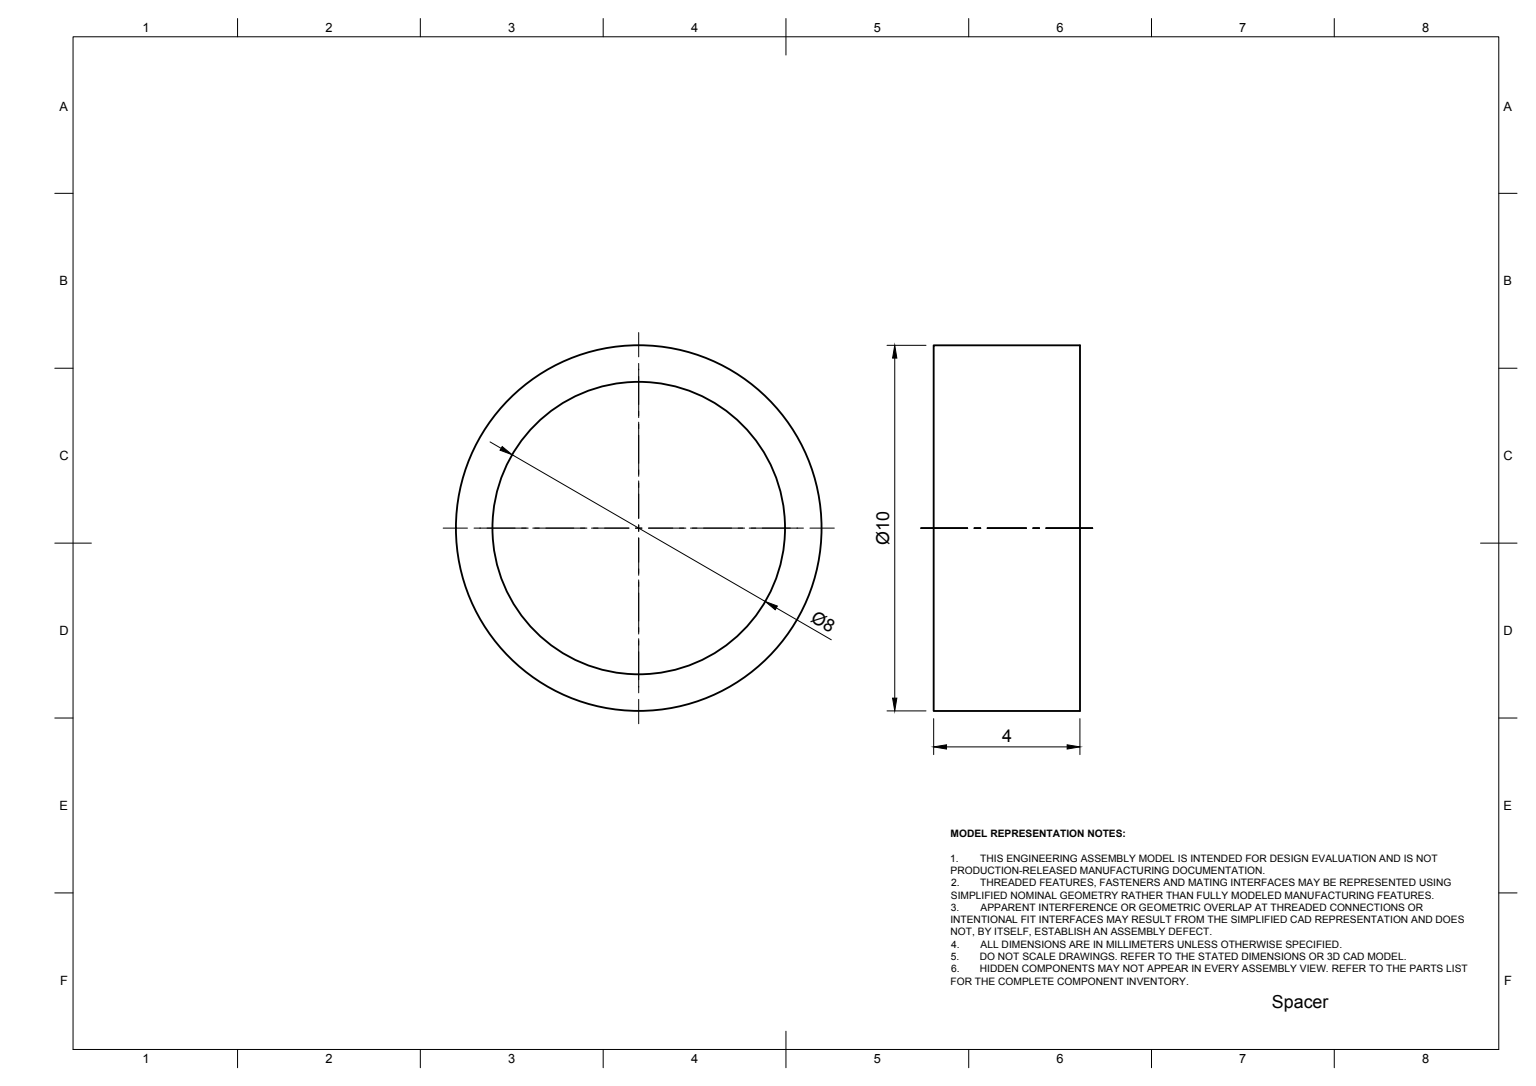
ISO-10303-21;
HEADER;
/* Generated by software containing ST-Developer
 * from STEP Tools, Inc. (www.steptools.com) 
 */

FILE_DESCRIPTION(
/* description */ (''),
/* implementation_level */ '2;1');

FILE_NAME(
/* name */ 'Spacer.step',
/* time_stamp */ '2026-10-04T12:17:52-07:00',
/* author */ (''),
/* organization */ (''),
/* preprocessor_version */ 'ST-DEVELOPER v20.2',
/* originating_system */ 'Autodesk Translation Framework v15.15.0.0',
/* authorisation */ '');

FILE_SCHEMA (('AUTOMOTIVE_DESIGN { 1 0 10303 214 3 1 1 }'));
ENDSEC;

DATA;
#10=MECHANICAL_DESIGN_GEOMETRIC_PRESENTATION_REPRESENTATION('',(#70),#1602);
#54=SHAPE_REPRESENTATION_RELATIONSHIP('SRR','None',#1641,#62);
#62=ADVANCED_BREP_SHAPE_REPRESENTATION('',(#78),#1601);
#70=STYLED_ITEM('',(#1684),#78);
#78=MANIFOLD_SOLID_BREP('Body1',#781);
#91=FACE_BOUND('',#260,.T.);
#92=FACE_BOUND('',#262,.T.);
#129=CIRCLE('',#960,4.);
#130=CIRCLE('',#961,4.);
#131=CIRCLE('',#963,5.);
#132=CIRCLE('',#964,5.);
#153=CYLINDRICAL_SURFACE('',#959,4.);
#154=CYLINDRICAL_SURFACE('',#962,5.);
#198=FACE_OUTER_BOUND('',#257,.T.);
#199=FACE_OUTER_BOUND('',#258,.T.);
#200=FACE_OUTER_BOUND('',#259,.T.);
#201=FACE_OUTER_BOUND('',#261,.T.);
#257=EDGE_LOOP('',(#690,#691,#692,#693));
#258=EDGE_LOOP('',(#694,#695,#696,#697));
#259=EDGE_LOOP('',(#698));
#260=EDGE_LOOP('',(#699));
#261=EDGE_LOOP('',(#700));
#262=EDGE_LOOP('',(#701));
#310=LINE('',#1565,#359);
#311=LINE('',#1571,#360);
#359=VECTOR('',#1202,4.);
#360=VECTOR('',#1209,5.);
#419=VERTEX_POINT('',#1562);
#420=VERTEX_POINT('',#1564);
#421=VERTEX_POINT('',#1568);
#422=VERTEX_POINT('',#1570);
#510=EDGE_CURVE('',#419,#419,#129,.T.);
#511=EDGE_CURVE('',#419,#420,#310,.T.);
#512=EDGE_CURVE('',#420,#420,#130,.T.);
#513=EDGE_CURVE('',#421,#421,#131,.T.);
#514=EDGE_CURVE('',#421,#422,#311,.T.);
#515=EDGE_CURVE('',#422,#422,#132,.T.);
#690=ORIENTED_EDGE('',*,*,#510,.T.);
#691=ORIENTED_EDGE('',*,*,#511,.T.);
#692=ORIENTED_EDGE('',*,*,#512,.F.);
#693=ORIENTED_EDGE('',*,*,#511,.F.);
#694=ORIENTED_EDGE('',*,*,#513,.F.);
#695=ORIENTED_EDGE('',*,*,#514,.T.);
#696=ORIENTED_EDGE('',*,*,#515,.T.);
#697=ORIENTED_EDGE('',*,*,#514,.F.);
#698=ORIENTED_EDGE('',*,*,#513,.T.);
#699=ORIENTED_EDGE('',*,*,#512,.T.);
#700=ORIENTED_EDGE('',*,*,#515,.F.);
#701=ORIENTED_EDGE('',*,*,#510,.F.);
#725=PLANE('',#965);
#726=PLANE('',#966);
#770=ADVANCED_FACE('',(#198),#153,.F.);
#771=ADVANCED_FACE('',(#199),#154,.T.);
#772=ADVANCED_FACE('',(#200,#91),#725,.T.);
#773=ADVANCED_FACE('',(#201,#92),#726,.F.);
#781=CLOSED_SHELL('',(#770,#771,#772,#773));
#958=AXIS2_PLACEMENT_3D('',#1560,#1196,#1197);
#959=AXIS2_PLACEMENT_3D('',#1561,#1198,#1199);
#960=AXIS2_PLACEMENT_3D('',#1563,#1200,#1201);
#961=AXIS2_PLACEMENT_3D('',#1566,#1203,#1204);
#962=AXIS2_PLACEMENT_3D('',#1567,#1205,#1206);
#963=AXIS2_PLACEMENT_3D('',#1569,#1207,#1208);
#964=AXIS2_PLACEMENT_3D('',#1572,#1210,#1211);
#965=AXIS2_PLACEMENT_3D('',#1573,#1212,#1213);
#966=AXIS2_PLACEMENT_3D('',#1574,#1214,#1215);
#1196=DIRECTION('axis',(0.,0.,1.));
#1197=DIRECTION('refdir',(1.,0.,0.));
#1198=DIRECTION('center_axis',(0.,-1.,0.));
#1199=DIRECTION('ref_axis',(1.,0.,0.));
#1200=DIRECTION('center_axis',(0.,1.,0.));
#1201=DIRECTION('ref_axis',(1.,0.,0.));
#1202=DIRECTION('',(0.,-1.,0.));
#1203=DIRECTION('center_axis',(0.,1.,0.));
#1204=DIRECTION('ref_axis',(1.,0.,0.));
#1205=DIRECTION('center_axis',(0.,-1.,0.));
#1206=DIRECTION('ref_axis',(1.,0.,0.));
#1207=DIRECTION('center_axis',(0.,-1.,0.));
#1208=DIRECTION('ref_axis',(1.,0.,0.));
#1209=DIRECTION('',(0.,1.,0.));
#1210=DIRECTION('center_axis',(0.,-1.,0.));
#1211=DIRECTION('ref_axis',(1.,0.,0.));
#1212=DIRECTION('center_axis',(0.,-1.,0.));
#1213=DIRECTION('ref_axis',(1.,0.,0.));
#1214=DIRECTION('center_axis',(0.,-1.,0.));
#1215=DIRECTION('ref_axis',(1.,0.,0.));
#1560=CARTESIAN_POINT('',(0.,0.,0.));
#1561=CARTESIAN_POINT('Origin',(23.8627874897787,4.,50.));
#1562=CARTESIAN_POINT('',(19.8627874897787,4.,50.));
#1563=CARTESIAN_POINT('Origin',(23.8627874897787,4.,50.));
#1564=CARTESIAN_POINT('',(19.8627874897787,5.55111512312578E-16,50.));
#1565=CARTESIAN_POINT('',(19.8627874897787,4.,50.));
#1566=CARTESIAN_POINT('Origin',(23.8627874897787,5.55111512312578E-16,50.));
#1567=CARTESIAN_POINT('Origin',(23.8627874897787,4.,50.));
#1568=CARTESIAN_POINT('',(18.8627874897787,5.55111512312578E-16,50.));
#1569=CARTESIAN_POINT('Origin',(23.8627874897787,5.55111512312578E-16,50.));
#1570=CARTESIAN_POINT('',(18.8627874897787,4.,50.));
#1571=CARTESIAN_POINT('',(18.8627874897787,4.,50.));
#1572=CARTESIAN_POINT('Origin',(23.8627874897787,4.,50.));
#1573=CARTESIAN_POINT('Origin',(23.8627874897787,5.55111512312578E-16,50.));
#1574=CARTESIAN_POINT('Origin',(23.8627874897787,4.,50.));
#1591=UNCERTAINTY_MEASURE_WITH_UNIT(LENGTH_MEASURE(0.01),#1603,
'DISTANCE_ACCURACY_VALUE',
'Maximum model space distance between geometric entities at asserted c
onnectivities');
#1592=UNCERTAINTY_MEASURE_WITH_UNIT(LENGTH_MEASURE(0.01),#1603,
'DISTANCE_ACCURACY_VALUE',
'Maximum model space distance between geometric entities at asserted c
onnectivities');
#1601=(
GEOMETRIC_REPRESENTATION_CONTEXT(3)
GLOBAL_UNCERTAINTY_ASSIGNED_CONTEXT((#1591))
GLOBAL_UNIT_ASSIGNED_CONTEXT((#1603,#1605,#1606))
REPRESENTATION_CONTEXT('','3D')
);
#1602=(
GEOMETRIC_REPRESENTATION_CONTEXT(3)
GLOBAL_UNCERTAINTY_ASSIGNED_CONTEXT((#1592))
GLOBAL_UNIT_ASSIGNED_CONTEXT((#1603,#1605,#1606))
REPRESENTATION_CONTEXT('','3D')
);
#1603=(
LENGTH_UNIT()
NAMED_UNIT(*)
SI_UNIT(.MILLI.,.METRE.)
);
#1605=(
NAMED_UNIT(*)
PLANE_ANGLE_UNIT()
SI_UNIT($,.RADIAN.)
);
#1606=(
NAMED_UNIT(*)
SI_UNIT($,.STERADIAN.)
SOLID_ANGLE_UNIT()
);
#1615=SHAPE_DEFINITION_REPRESENTATION(#1624,#1641);
#1624=PRODUCT_DEFINITION_SHAPE('',$,#1651);
#1641=SHAPE_REPRESENTATION('',(#958),#1601);
#1642=PRODUCT_DEFINITION_CONTEXT('part definition',#1671,'design');
#1651=PRODUCT_DEFINITION('spacer','Spacer',#1660,#1642);
#1660=PRODUCT_DEFINITION_FORMATION('',$,#1681);
#1671=APPLICATION_CONTEXT(
'Core Data for Automotive Mechanical Design Process');
#1672=PRODUCT_CONTEXT('part definition',#1671,'mechanical');
#1681=PRODUCT('spacer','Spacer',$,(#1672));
#1684=PRESENTATION_STYLE_ASSIGNMENT((#1688));
#1688=SURFACE_STYLE_USAGE(.BOTH.,#1692);
#1692=SURFACE_SIDE_STYLE('',(#1696));
#1696=SURFACE_STYLE_FILL_AREA(#1700);
#1700=FILL_AREA_STYLE('Opaque(160,160,160)',(#1704));
#1704=FILL_AREA_STYLE_COLOUR('Opaque(160,160,160)',#1708);
#1708=COLOUR_RGB('Opaque(160,160,160)', 0.66274510, 0.83137255, 0.94901961);
ENDSEC;
END-ISO-10303-21;
